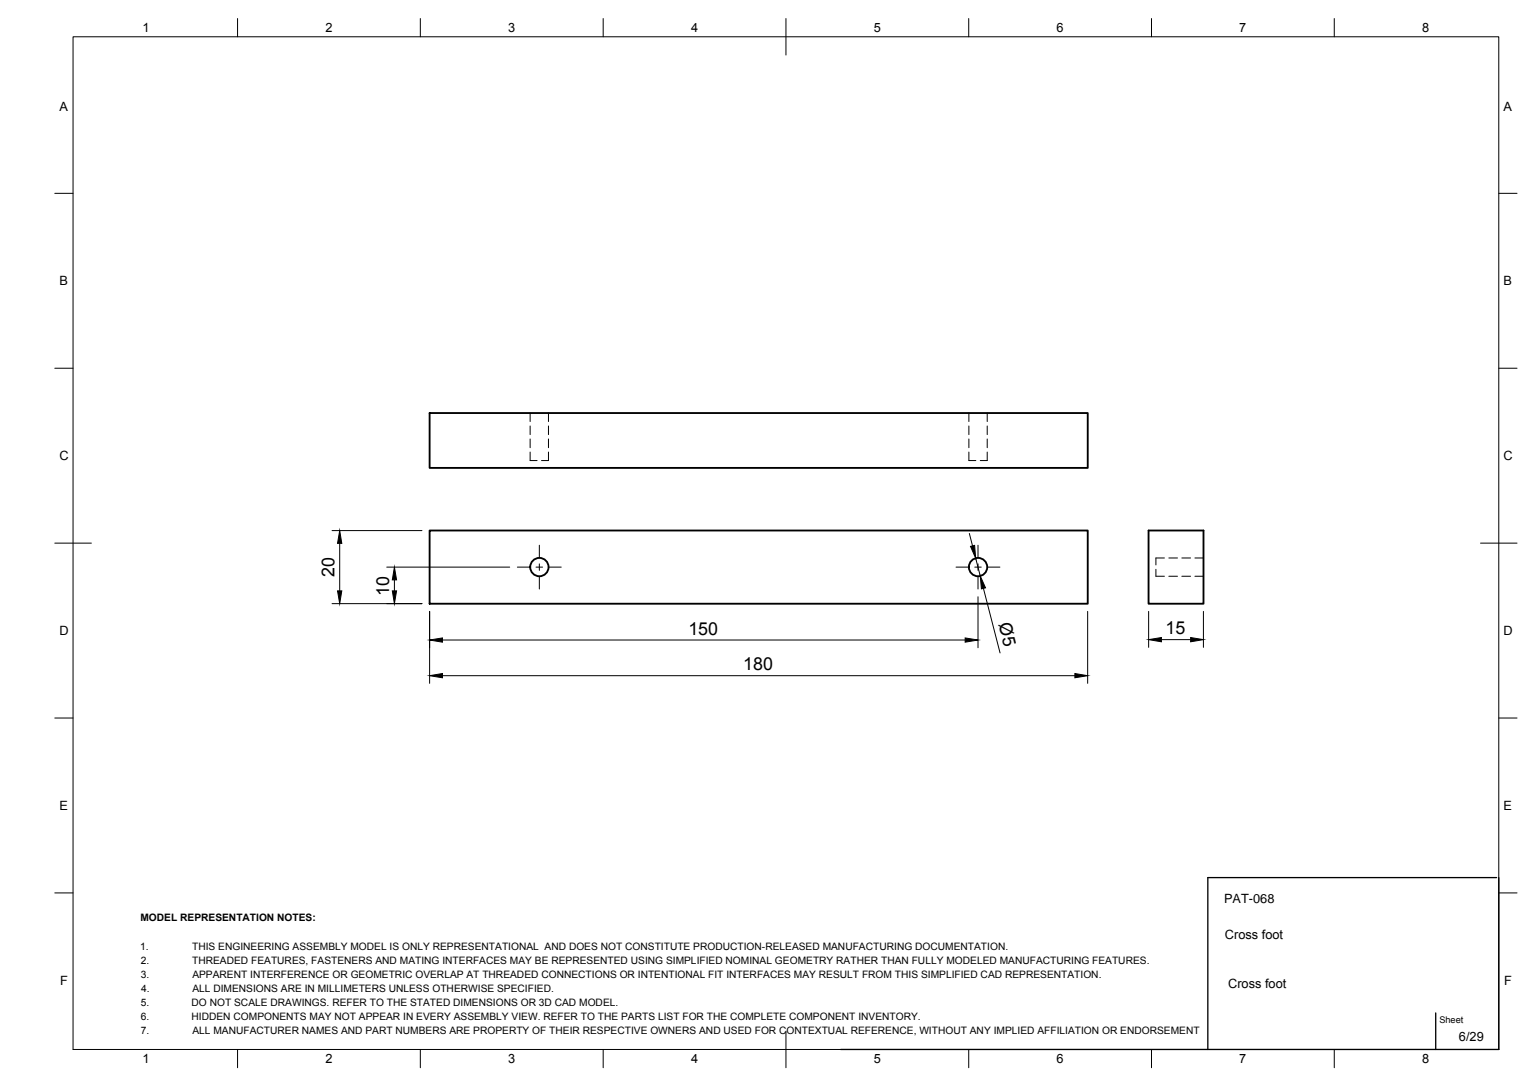
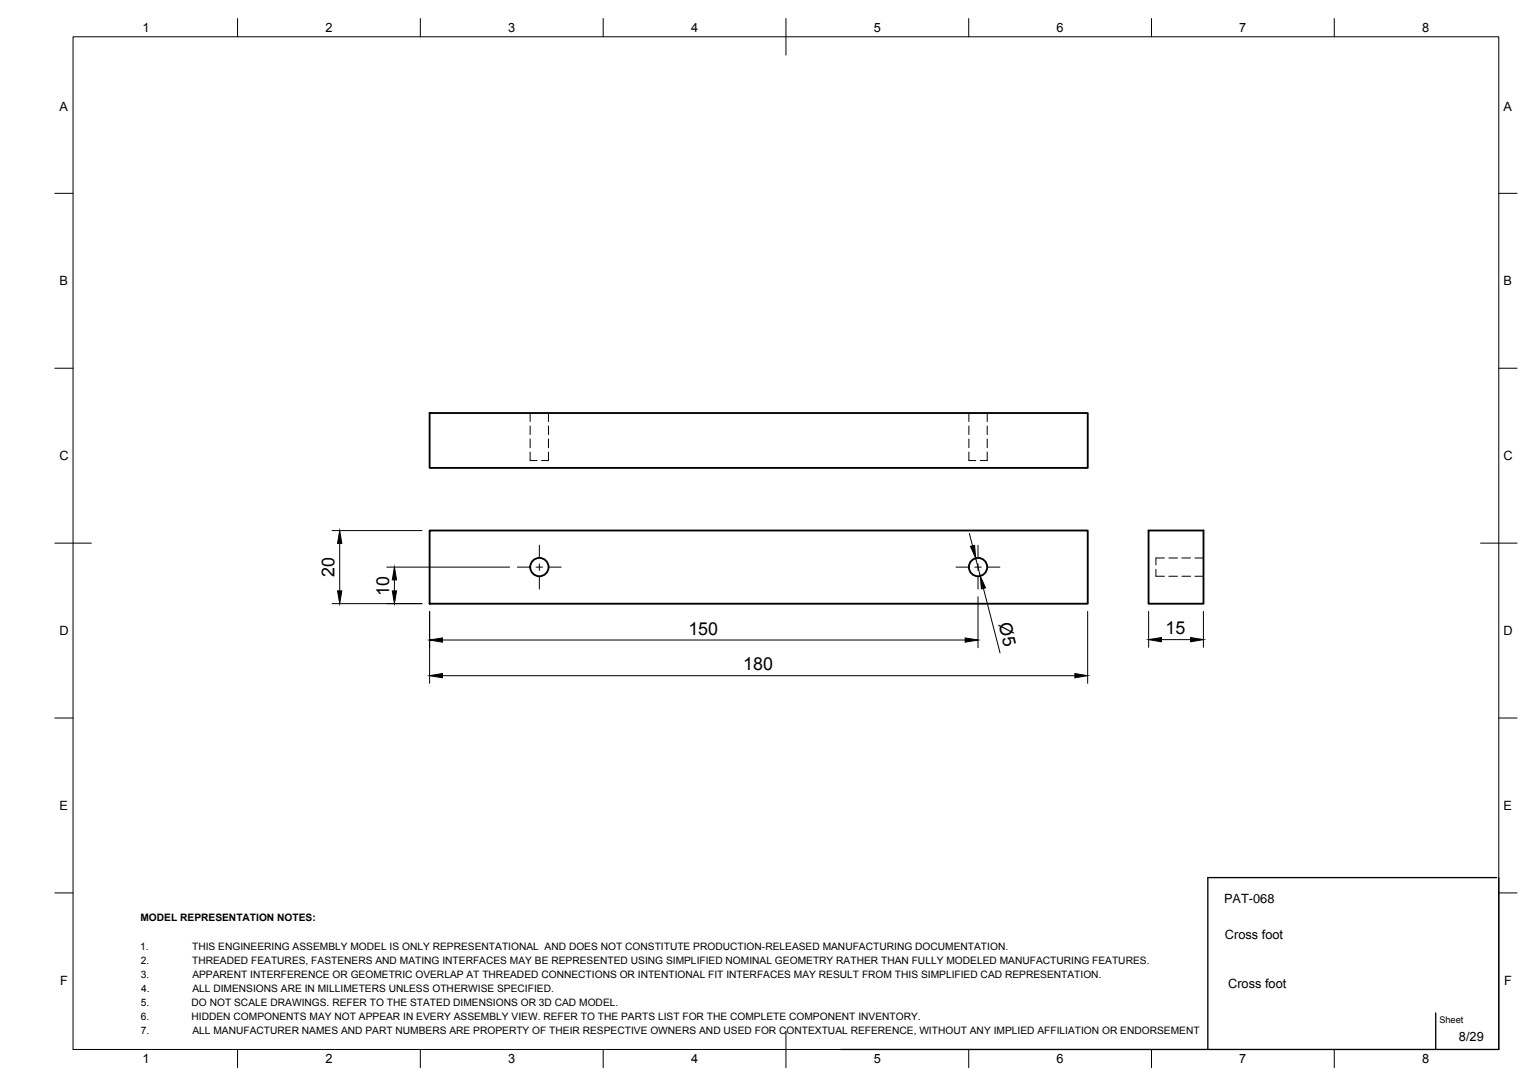
ISO-10303-21;
HEADER;
/* Generated by software containing ST-Developer
 * from STEP Tools, Inc. (www.steptools.com) 
 */

FILE_DESCRIPTION(
/* description */ ('Line shaft on three pillow blocks'),
/* implementation_level */ '2;1');

FILE_NAME(
/* name */ 'Cross foot.step',
/* time_stamp */ '2026-10-27T10:49:19-07:00',
/* author */ (''),
/* organization */ (''),
/* preprocessor_version */ 'ST-DEVELOPER v20.2',
/* originating_system */ 'Autodesk Translation Framework v15.17.0.0',
/* authorisation */ '');

FILE_SCHEMA (('AUTOMOTIVE_DESIGN { 1 0 10303 214 3 1 1 }'));
ENDSEC;

DATA;
#10=MECHANICAL_DESIGN_GEOMETRIC_PRESENTATION_REPRESENTATION('',(#339),#8377);
#285=SHAPE_REPRESENTATION_RELATIONSHIP('SRR','None',#8500,#312);
#312=ADVANCED_BREP_SHAPE_REPRESENTATION('',(#367),#8349);
#339=STYLED_ITEM('',(#8732),#367);
#367=MANIFOLD_SOLID_BREP('Body1',#4325);
#411=FACE_BOUND('',#951,.T.);
#412=FACE_BOUND('',#952,.T.);
#494=PLANE('',#4696);
#495=PLANE('',#4700);
#496=PLANE('',#4701);
#497=PLANE('',#4702);
#498=PLANE('',#4703);
#499=PLANE('',#4704);
#500=PLANE('',#4705);
#501=PLANE('',#4706);
#670=FACE_OUTER_BOUND('',#942,.T.);
#671=FACE_OUTER_BOUND('',#943,.T.);
#672=FACE_OUTER_BOUND('',#944,.T.);
#673=FACE_OUTER_BOUND('',#945,.T.);
#674=FACE_OUTER_BOUND('',#946,.T.);
#675=FACE_OUTER_BOUND('',#947,.T.);
#676=FACE_OUTER_BOUND('',#948,.T.);
#677=FACE_OUTER_BOUND('',#949,.T.);
#678=FACE_OUTER_BOUND('',#950,.T.);
#679=FACE_OUTER_BOUND('',#953,.T.);
#942=EDGE_LOOP('',(#3033,#3034,#3035,#3036));
#943=EDGE_LOOP('',(#3037));
#944=EDGE_LOOP('',(#3038,#3039,#3040,#3041));
#945=EDGE_LOOP('',(#3042));
#946=EDGE_LOOP('',(#3043,#3044,#3045,#3046));
#947=EDGE_LOOP('',(#3047,#3048,#3049,#3050));
#948=EDGE_LOOP('',(#3051,#3052,#3053,#3054));
#949=EDGE_LOOP('',(#3055,#3056,#3057,#3058));
#950=EDGE_LOOP('',(#3059,#3060,#3061,#3062));
#951=EDGE_LOOP('',(#3063));
#952=EDGE_LOOP('',(#3064));
#953=EDGE_LOOP('',(#3065,#3066,#3067,#3068));
#1277=LINE('',#6559,#1604);
#1278=LINE('',#6566,#1605);
#1279=LINE('',#6572,#1606);
#1280=LINE('',#6574,#1607);
#1281=LINE('',#6576,#1608);
#1282=LINE('',#6577,#1609);
#1283=LINE('',#6580,#1610);
#1284=LINE('',#6582,#1611);
#1285=LINE('',#6583,#1612);
#1286=LINE('',#6586,#1613);
#1287=LINE('',#6588,#1614);
#1288=LINE('',#6589,#1615);
#1289=LINE('',#6591,#1616);
#1290=LINE('',#6592,#1617);
#1604=VECTOR('',#5254,0.25);
#1605=VECTOR('',#5263,0.25);
#1606=VECTOR('',#5270,1.);
#1607=VECTOR('',#5271,1.);
#1608=VECTOR('',#5272,1.);
#1609=VECTOR('',#5273,1.);
#1610=VECTOR('',#5276,1.);
#1611=VECTOR('',#5277,1.);
#1612=VECTOR('',#5278,1.);
#1613=VECTOR('',#5281,1.);
#1614=VECTOR('',#5282,1.);
#1615=VECTOR('',#5283,1.);
#1616=VECTOR('',#5286,1.);
#1617=VECTOR('',#5287,1.);
#1929=CIRCLE('',#4694,0.25);
#1930=CIRCLE('',#4695,0.25);
#1931=CIRCLE('',#4698,0.25);
#1932=CIRCLE('',#4699,0.25);
#2096=VERTEX_POINT('',#6556);
#2097=VERTEX_POINT('',#6558);
#2098=VERTEX_POINT('',#6563);
#2099=VERTEX_POINT('',#6565);
#2100=VERTEX_POINT('',#6570);
#2101=VERTEX_POINT('',#6571);
#2102=VERTEX_POINT('',#6573);
#2103=VERTEX_POINT('',#6575);
#2104=VERTEX_POINT('',#6579);
#2105=VERTEX_POINT('',#6581);
#2106=VERTEX_POINT('',#6585);
#2107=VERTEX_POINT('',#6587);
#2465=EDGE_CURVE('',#2096,#2096,#1929,.T.);
#2466=EDGE_CURVE('',#2096,#2097,#1277,.T.);
#2467=EDGE_CURVE('',#2097,#2097,#1930,.T.);
#2468=EDGE_CURVE('',#2098,#2098,#1931,.T.);
#2469=EDGE_CURVE('',#2098,#2099,#1278,.T.);
#2470=EDGE_CURVE('',#2099,#2099,#1932,.T.);
#2471=EDGE_CURVE('',#2100,#2101,#1279,.T.);
#2472=EDGE_CURVE('',#2101,#2102,#1280,.T.);
#2473=EDGE_CURVE('',#2103,#2102,#1281,.T.);
#2474=EDGE_CURVE('',#2100,#2103,#1282,.T.);
#2475=EDGE_CURVE('',#2104,#2100,#1283,.T.);
#2476=EDGE_CURVE('',#2105,#2103,#1284,.T.);
#2477=EDGE_CURVE('',#2104,#2105,#1285,.T.);
#2478=EDGE_CURVE('',#2106,#2104,#1286,.T.);
#2479=EDGE_CURVE('',#2107,#2105,#1287,.T.);
#2480=EDGE_CURVE('',#2106,#2107,#1288,.T.);
#2481=EDGE_CURVE('',#2101,#2106,#1289,.T.);
#2482=EDGE_CURVE('',#2102,#2107,#1290,.T.);
#3033=ORIENTED_EDGE('',*,*,#2465,.F.);
#3034=ORIENTED_EDGE('',*,*,#2466,.T.);
#3035=ORIENTED_EDGE('',*,*,#2467,.F.);
#3036=ORIENTED_EDGE('',*,*,#2466,.F.);
#3037=ORIENTED_EDGE('',*,*,#2465,.T.);
#3038=ORIENTED_EDGE('',*,*,#2468,.F.);
#3039=ORIENTED_EDGE('',*,*,#2469,.T.);
#3040=ORIENTED_EDGE('',*,*,#2470,.F.);
#3041=ORIENTED_EDGE('',*,*,#2469,.F.);
#3042=ORIENTED_EDGE('',*,*,#2468,.T.);
#3043=ORIENTED_EDGE('',*,*,#2471,.T.);
#3044=ORIENTED_EDGE('',*,*,#2472,.T.);
#3045=ORIENTED_EDGE('',*,*,#2473,.F.);
#3046=ORIENTED_EDGE('',*,*,#2474,.F.);
#3047=ORIENTED_EDGE('',*,*,#2475,.T.);
#3048=ORIENTED_EDGE('',*,*,#2474,.T.);
#3049=ORIENTED_EDGE('',*,*,#2476,.F.);
#3050=ORIENTED_EDGE('',*,*,#2477,.F.);
#3051=ORIENTED_EDGE('',*,*,#2478,.T.);
#3052=ORIENTED_EDGE('',*,*,#2477,.T.);
#3053=ORIENTED_EDGE('',*,*,#2479,.F.);
#3054=ORIENTED_EDGE('',*,*,#2480,.F.);
#3055=ORIENTED_EDGE('',*,*,#2481,.T.);
#3056=ORIENTED_EDGE('',*,*,#2480,.T.);
#3057=ORIENTED_EDGE('',*,*,#2482,.F.);
#3058=ORIENTED_EDGE('',*,*,#2472,.F.);
#3059=ORIENTED_EDGE('',*,*,#2482,.T.);
#3060=ORIENTED_EDGE('',*,*,#2479,.T.);
#3061=ORIENTED_EDGE('',*,*,#2476,.T.);
#3062=ORIENTED_EDGE('',*,*,#2473,.T.);
#3063=ORIENTED_EDGE('',*,*,#2467,.T.);
#3064=ORIENTED_EDGE('',*,*,#2470,.T.);
#3065=ORIENTED_EDGE('',*,*,#2481,.F.);
#3066=ORIENTED_EDGE('',*,*,#2471,.F.);
#3067=ORIENTED_EDGE('',*,*,#2475,.F.);
#3068=ORIENTED_EDGE('',*,*,#2478,.F.);
#4011=CYLINDRICAL_SURFACE('',#4693,0.25);
#4012=CYLINDRICAL_SURFACE('',#4697,0.25);
#4088=ADVANCED_FACE('',(#670),#4011,.F.);
#4089=ADVANCED_FACE('',(#671),#494,.T.);
#4090=ADVANCED_FACE('',(#672),#4012,.F.);
#4091=ADVANCED_FACE('',(#673),#495,.T.);
#4092=ADVANCED_FACE('',(#674),#496,.T.);
#4093=ADVANCED_FACE('',(#675),#497,.T.);
#4094=ADVANCED_FACE('',(#676),#498,.T.);
#4095=ADVANCED_FACE('',(#677),#499,.T.);
#4096=ADVANCED_FACE('',(#678,#411,#412),#500,.T.);
#4097=ADVANCED_FACE('',(#679),#501,.F.);
#4325=CLOSED_SHELL('',(#4088,#4089,#4090,#4091,#4092,#4093,#4094,#4095,
#4096,#4097));
#4692=AXIS2_PLACEMENT_3D('',#6554,#5248,#5249);
#4693=AXIS2_PLACEMENT_3D('',#6555,#5250,#5251);
#4694=AXIS2_PLACEMENT_3D('',#6557,#5252,#5253);
#4695=AXIS2_PLACEMENT_3D('',#6560,#5255,#5256);
#4696=AXIS2_PLACEMENT_3D('',#6561,#5257,#5258);
#4697=AXIS2_PLACEMENT_3D('',#6562,#5259,#5260);
#4698=AXIS2_PLACEMENT_3D('',#6564,#5261,#5262);
#4699=AXIS2_PLACEMENT_3D('',#6567,#5264,#5265);
#4700=AXIS2_PLACEMENT_3D('',#6568,#5266,#5267);
#4701=AXIS2_PLACEMENT_3D('',#6569,#5268,#5269);
#4702=AXIS2_PLACEMENT_3D('',#6578,#5274,#5275);
#4703=AXIS2_PLACEMENT_3D('',#6584,#5279,#5280);
#4704=AXIS2_PLACEMENT_3D('',#6590,#5284,#5285);
#4705=AXIS2_PLACEMENT_3D('',#6593,#5288,#5289);
#4706=AXIS2_PLACEMENT_3D('',#6594,#5290,#5291);
#5248=DIRECTION('axis',(0.,0.,1.));
#5249=DIRECTION('refdir',(1.,0.,0.));
#5250=DIRECTION('center_axis',(0.,0.,1.));
#5251=DIRECTION('ref_axis',(1.,0.,0.));
#5252=DIRECTION('center_axis',(0.,0.,1.));
#5253=DIRECTION('ref_axis',(1.,0.,0.));
#5254=DIRECTION('',(0.,0.,1.));
#5255=DIRECTION('center_axis',(0.,0.,-1.));
#5256=DIRECTION('ref_axis',(1.,0.,0.));
#5257=DIRECTION('center_axis',(0.,0.,1.));
#5258=DIRECTION('ref_axis',(1.,0.,0.));
#5259=DIRECTION('center_axis',(0.,0.,1.));
#5260=DIRECTION('ref_axis',(1.,0.,0.));
#5261=DIRECTION('center_axis',(0.,0.,1.));
#5262=DIRECTION('ref_axis',(1.,0.,0.));
#5263=DIRECTION('',(0.,0.,1.));
#5264=DIRECTION('center_axis',(0.,0.,-1.));
#5265=DIRECTION('ref_axis',(1.,0.,0.));
#5266=DIRECTION('center_axis',(0.,0.,1.));
#5267=DIRECTION('ref_axis',(1.,0.,0.));
#5268=DIRECTION('center_axis',(0.,1.,0.));
#5269=DIRECTION('ref_axis',(-1.,0.,0.));
#5270=DIRECTION('',(-1.,0.,0.));
#5271=DIRECTION('',(0.,0.,1.));
#5272=DIRECTION('',(-1.,0.,0.));
#5273=DIRECTION('',(0.,0.,1.));
#5274=DIRECTION('center_axis',(1.,0.,0.));
#5275=DIRECTION('ref_axis',(0.,1.,0.));
#5276=DIRECTION('',(0.,1.,0.));
#5277=DIRECTION('',(0.,1.,0.));
#5278=DIRECTION('',(0.,0.,1.));
#5279=DIRECTION('center_axis',(0.,-1.,0.));
#5280=DIRECTION('ref_axis',(1.,0.,0.));
#5281=DIRECTION('',(1.,0.,0.));
#5282=DIRECTION('',(1.,0.,0.));
#5283=DIRECTION('',(0.,0.,1.));
#5284=DIRECTION('center_axis',(-1.,0.,0.));
#5285=DIRECTION('ref_axis',(0.,-1.,0.));
#5286=DIRECTION('',(0.,-1.,0.));
#5287=DIRECTION('',(0.,-1.,0.));
#5288=DIRECTION('center_axis',(0.,0.,1.));
#5289=DIRECTION('ref_axis',(1.,0.,0.));
#5290=DIRECTION('center_axis',(0.,0.,1.));
#5291=DIRECTION('ref_axis',(1.,0.,0.));
#6554=CARTESIAN_POINT('',(0.,0.,0.));
#6555=CARTESIAN_POINT('Origin',(-6.,-3.,-1.3));
#6556=CARTESIAN_POINT('',(-6.25,-3.,-1.3));
#6557=CARTESIAN_POINT('Origin',(-6.,-3.,-1.3));
#6558=CARTESIAN_POINT('',(-6.25,-3.,0.));
#6559=CARTESIAN_POINT('',(-6.25,-3.,-1.3));
#6560=CARTESIAN_POINT('Origin',(-6.,-3.,0.));
#6561=CARTESIAN_POINT('Origin',(-6.,-3.,-1.3));
#6562=CARTESIAN_POINT('Origin',(6.,-3.,-1.3));
#6563=CARTESIAN_POINT('',(5.75,-3.,-1.3));
#6564=CARTESIAN_POINT('Origin',(6.,-3.,-1.3));
#6565=CARTESIAN_POINT('',(5.75,-3.,0.));
#6566=CARTESIAN_POINT('',(5.75,-3.,-1.3));
#6567=CARTESIAN_POINT('Origin',(6.,-3.,0.));
#6568=CARTESIAN_POINT('Origin',(6.,-3.,-1.3));
#6569=CARTESIAN_POINT('Origin',(9.,-2.,-1.5));
#6570=CARTESIAN_POINT('',(9.,-2.,-1.5));
#6571=CARTESIAN_POINT('',(-9.,-2.,-1.5));
#6572=CARTESIAN_POINT('',(9.,-2.,-1.5));
#6573=CARTESIAN_POINT('',(-9.,-2.,0.));
#6574=CARTESIAN_POINT('',(-9.,-2.,-1.5));
#6575=CARTESIAN_POINT('',(9.,-2.,0.));
#6576=CARTESIAN_POINT('',(9.,-2.,0.));
#6577=CARTESIAN_POINT('',(9.,-2.,-1.5));
#6578=CARTESIAN_POINT('Origin',(9.,-4.,-1.5));
#6579=CARTESIAN_POINT('',(9.,-4.,-1.5));
#6580=CARTESIAN_POINT('',(9.,-4.,-1.5));
#6581=CARTESIAN_POINT('',(9.,-4.,0.));
#6582=CARTESIAN_POINT('',(9.,-4.,0.));
#6583=CARTESIAN_POINT('',(9.,-4.,-1.5));
#6584=CARTESIAN_POINT('Origin',(-9.,-4.,-1.5));
#6585=CARTESIAN_POINT('',(-9.,-4.,-1.5));
#6586=CARTESIAN_POINT('',(-9.,-4.,-1.5));
#6587=CARTESIAN_POINT('',(-9.,-4.,0.));
#6588=CARTESIAN_POINT('',(-9.,-4.,0.));
#6589=CARTESIAN_POINT('',(-9.,-4.,-1.5));
#6590=CARTESIAN_POINT('Origin',(-9.,-2.,-1.5));
#6591=CARTESIAN_POINT('',(-9.,-2.,-1.5));
#6592=CARTESIAN_POINT('',(-9.,-2.,0.));
#6593=CARTESIAN_POINT('Origin',(0.,-3.,0.));
#6594=CARTESIAN_POINT('Origin',(0.,-3.,-1.5));
#8317=UNCERTAINTY_MEASURE_WITH_UNIT(LENGTH_MEASURE(0.001),#8378,
'DISTANCE_ACCURACY_VALUE',
'Maximum model space distance between geometric entities at asserted c
onnectivities');
#8345=UNCERTAINTY_MEASURE_WITH_UNIT(LENGTH_MEASURE(0.001),#8378,
'DISTANCE_ACCURACY_VALUE',
'Maximum model space distance between geometric entities at asserted c
onnectivities');
#8349=(
GEOMETRIC_REPRESENTATION_CONTEXT(3)
GLOBAL_UNCERTAINTY_ASSIGNED_CONTEXT((#8317))
GLOBAL_UNIT_ASSIGNED_CONTEXT((#8378,#8380,#8381))
REPRESENTATION_CONTEXT('','3D')
);
#8377=(
GEOMETRIC_REPRESENTATION_CONTEXT(3)
GLOBAL_UNCERTAINTY_ASSIGNED_CONTEXT((#8345))
GLOBAL_UNIT_ASSIGNED_CONTEXT((#8378,#8380,#8381))
REPRESENTATION_CONTEXT('','3D')
);
#8378=(
LENGTH_UNIT()
NAMED_UNIT(*)
SI_UNIT(.CENTI.,.METRE.)
);
#8380=(
NAMED_UNIT(*)
PLANE_ANGLE_UNIT()
SI_UNIT($,.RADIAN.)
);
#8381=(
NAMED_UNIT(*)
SI_UNIT($,.STERADIAN.)
SOLID_ANGLE_UNIT()
);
#8385=SHAPE_DEFINITION_REPRESENTATION(#8416,#8500);
#8416=PRODUCT_DEFINITION_SHAPE('',$,#8532);
#8500=SHAPE_REPRESENTATION('',(#4692),#8349);
#8528=PRODUCT_DEFINITION_CONTEXT('part definition',#8623,'design');
#8532=PRODUCT_DEFINITION('Cross foot','Cross foot',#8563,#8528);
#8563=PRODUCT_DEFINITION_FORMATION('',$,#8628);
#8623=APPLICATION_CONTEXT(
'Core Data for Automotive Mechanical Design Process');
#8624=PRODUCT_CONTEXT('part definition',#8623,'mechanical');
#8628=PRODUCT('Cross foot','Cross foot','Cross foot',(#8624));
#8726=COLOUR_RGB('Off White',0.89,0.88,0.83);
#8727=FILL_AREA_STYLE_COLOUR('',#8726);
#8728=FILL_AREA_STYLE('',(#8727));
#8729=SURFACE_STYLE_FILL_AREA(#8728);
#8730=SURFACE_SIDE_STYLE('',(#8729));
#8731=SURFACE_STYLE_USAGE(.BOTH.,#8730);
#8732=PRESENTATION_STYLE_ASSIGNMENT((#8731));
ENDSEC;
END-ISO-10303-21;
